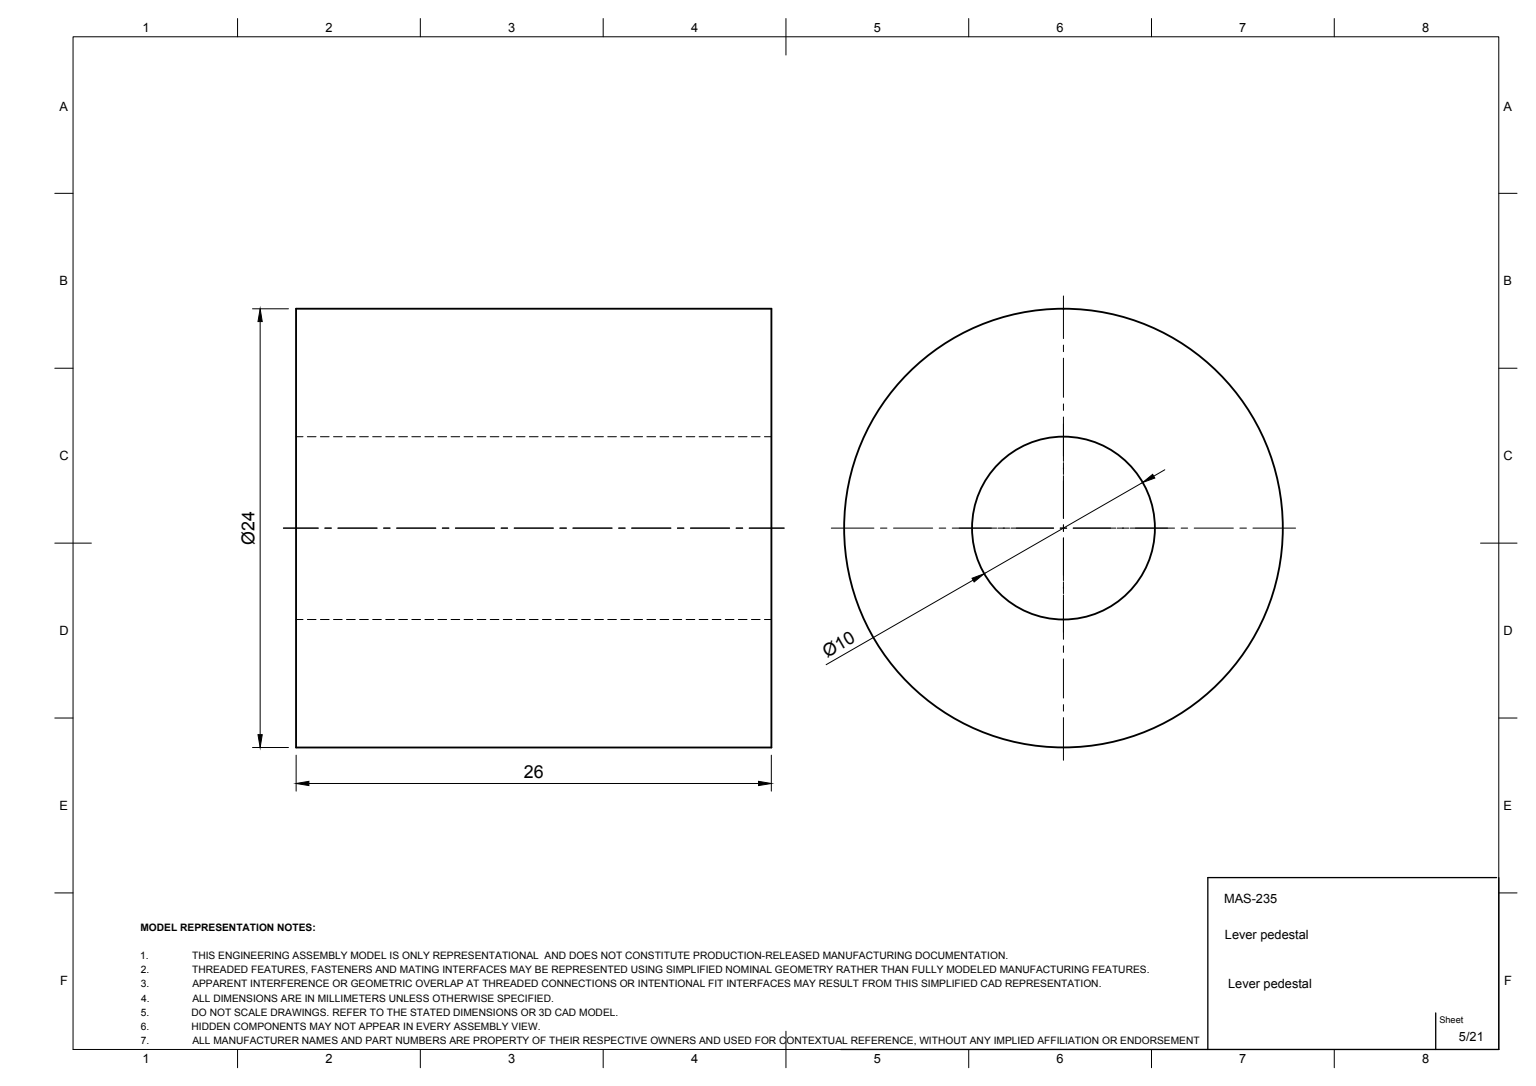
ISO-10303-21;
HEADER;
/* Generated by software containing ST-Developer
 * from STEP Tools, Inc. (www.steptools.com) 
 */

FILE_DESCRIPTION(
/* description */ ('Independent Whitworth quick-return mechanism. Crank radius40, ground-
center spacing80, lever180, connecting rod160, output guide X200. Nomi
nal stroke180 and long/short phase ratio2. Retained guide rods, replac
eable bearing sleeves and captured sliding shoe. No load or production
 rating assigned.'),
/* implementation_level */ '2;1');

FILE_NAME(
/* name */ 'Lever pedestal.step',
/* time_stamp */ '2026-11-09T18:22:56-08:00',
/* author */ (''),
/* organization */ (''),
/* preprocessor_version */ 'ST-DEVELOPER v20.2',
/* originating_system */ 'Autodesk Translation Framework v15.17.0.0',
/* authorisation */ '');

FILE_SCHEMA (('AUTOMOTIVE_DESIGN { 1 0 10303 214 3 1 1 }'));
ENDSEC;

DATA;
#10=MECHANICAL_DESIGN_GEOMETRIC_PRESENTATION_REPRESENTATION('',(#221),#4388);
#181=SHAPE_REPRESENTATION_RELATIONSHIP('SRR','None',#4480,#201);
#201=ADVANCED_BREP_SHAPE_REPRESENTATION('',(#241),#4370);
#221=STYLED_ITEM('',(#4588),#241);
#241=MANIFOLD_SOLID_BREP('Body1',#2326);
#265=FACE_BOUND('',#573,.T.);
#266=FACE_BOUND('',#575,.T.);
#327=PLANE('',#2595);
#328=PLANE('',#2596);
#417=FACE_OUTER_BOUND('',#570,.T.);
#418=FACE_OUTER_BOUND('',#571,.T.);
#419=FACE_OUTER_BOUND('',#572,.T.);
#420=FACE_OUTER_BOUND('',#574,.T.);
#570=EDGE_LOOP('',(#1642,#1643,#1644,#1645));
#571=EDGE_LOOP('',(#1646,#1647,#1648,#1649));
#572=EDGE_LOOP('',(#1650));
#573=EDGE_LOOP('',(#1651));
#574=EDGE_LOOP('',(#1652));
#575=EDGE_LOOP('',(#1653));
#775=LINE('',#3760,#914);
#776=LINE('',#3766,#915);
#914=VECTOR('',#2965,5.);
#915=VECTOR('',#2972,12.);
#1045=CIRCLE('',#2590,5.);
#1046=CIRCLE('',#2591,5.);
#1047=CIRCLE('',#2593,12.);
#1048=CIRCLE('',#2594,12.);
#1175=VERTEX_POINT('',#3757);
#1176=VERTEX_POINT('',#3759);
#1177=VERTEX_POINT('',#3763);
#1178=VERTEX_POINT('',#3765);
#1357=EDGE_CURVE('',#1175,#1175,#1045,.T.);
#1358=EDGE_CURVE('',#1175,#1176,#775,.T.);
#1359=EDGE_CURVE('',#1176,#1176,#1046,.T.);
#1360=EDGE_CURVE('',#1177,#1177,#1047,.T.);
#1361=EDGE_CURVE('',#1177,#1178,#776,.T.);
#1362=EDGE_CURVE('',#1178,#1178,#1048,.T.);
#1642=ORIENTED_EDGE('',*,*,#1357,.F.);
#1643=ORIENTED_EDGE('',*,*,#1358,.T.);
#1644=ORIENTED_EDGE('',*,*,#1359,.T.);
#1645=ORIENTED_EDGE('',*,*,#1358,.F.);
#1646=ORIENTED_EDGE('',*,*,#1360,.F.);
#1647=ORIENTED_EDGE('',*,*,#1361,.T.);
#1648=ORIENTED_EDGE('',*,*,#1362,.T.);
#1649=ORIENTED_EDGE('',*,*,#1361,.F.);
#1650=ORIENTED_EDGE('',*,*,#1360,.T.);
#1651=ORIENTED_EDGE('',*,*,#1357,.T.);
#1652=ORIENTED_EDGE('',*,*,#1362,.F.);
#1653=ORIENTED_EDGE('',*,*,#1359,.F.);
#2120=CYLINDRICAL_SURFACE('',#2589,5.);
#2121=CYLINDRICAL_SURFACE('',#2592,12.);
#2189=ADVANCED_FACE('',(#417),#2120,.F.);
#2190=ADVANCED_FACE('',(#418),#2121,.T.);
#2191=ADVANCED_FACE('',(#419,#265),#327,.T.);
#2192=ADVANCED_FACE('',(#420,#266),#328,.F.);
#2326=CLOSED_SHELL('',(#2189,#2190,#2191,#2192));
#2588=AXIS2_PLACEMENT_3D('',#3755,#2959,#2960);
#2589=AXIS2_PLACEMENT_3D('',#3756,#2961,#2962);
#2590=AXIS2_PLACEMENT_3D('',#3758,#2963,#2964);
#2591=AXIS2_PLACEMENT_3D('',#3761,#2966,#2967);
#2592=AXIS2_PLACEMENT_3D('',#3762,#2968,#2969);
#2593=AXIS2_PLACEMENT_3D('',#3764,#2970,#2971);
#2594=AXIS2_PLACEMENT_3D('',#3767,#2973,#2974);
#2595=AXIS2_PLACEMENT_3D('',#3768,#2975,#2976);
#2596=AXIS2_PLACEMENT_3D('',#3769,#2977,#2978);
#2959=DIRECTION('axis',(0.,0.,1.));
#2960=DIRECTION('refdir',(1.,0.,0.));
#2961=DIRECTION('center_axis',(0.,0.,1.));
#2962=DIRECTION('ref_axis',(1.,0.,0.));
#2963=DIRECTION('center_axis',(0.,0.,-1.));
#2964=DIRECTION('ref_axis',(1.,0.,0.));
#2965=DIRECTION('',(0.,0.,-1.));
#2966=DIRECTION('center_axis',(0.,0.,-1.));
#2967=DIRECTION('ref_axis',(1.,0.,0.));
#2968=DIRECTION('center_axis',(0.,0.,1.));
#2969=DIRECTION('ref_axis',(1.,0.,0.));
#2970=DIRECTION('center_axis',(0.,0.,1.));
#2971=DIRECTION('ref_axis',(1.,0.,0.));
#2972=DIRECTION('',(0.,0.,-1.));
#2973=DIRECTION('center_axis',(0.,0.,1.));
#2974=DIRECTION('ref_axis',(1.,0.,0.));
#2975=DIRECTION('center_axis',(0.,0.,1.));
#2976=DIRECTION('ref_axis',(1.,0.,0.));
#2977=DIRECTION('center_axis',(0.,0.,1.));
#2978=DIRECTION('ref_axis',(1.,0.,0.));
#3755=CARTESIAN_POINT('',(0.,0.,0.));
#3756=CARTESIAN_POINT('Origin',(0.,0.,0.));
#3757=CARTESIAN_POINT('',(-5.,-6.12323399573677E-16,26.));
#3758=CARTESIAN_POINT('Origin',(0.,0.,26.));
#3759=CARTESIAN_POINT('',(-5.,-6.12323399573677E-16,0.));
#3760=CARTESIAN_POINT('',(-5.,-6.12323399573677E-16,0.));
#3761=CARTESIAN_POINT('Origin',(0.,0.,0.));
#3762=CARTESIAN_POINT('Origin',(0.,0.,0.));
#3763=CARTESIAN_POINT('',(-12.,-1.46957615897682E-15,26.));
#3764=CARTESIAN_POINT('Origin',(0.,0.,26.));
#3765=CARTESIAN_POINT('',(-12.,-1.46957615897682E-15,0.));
#3766=CARTESIAN_POINT('',(-12.,-1.46957615897682E-15,0.));
#3767=CARTESIAN_POINT('Origin',(0.,0.,0.));
#3768=CARTESIAN_POINT('Origin',(0.,0.,26.));
#3769=CARTESIAN_POINT('Origin',(0.,0.,0.));
#4348=UNCERTAINTY_MEASURE_WITH_UNIT(LENGTH_MEASURE(0.01),#4389,
'DISTANCE_ACCURACY_VALUE',
'Maximum model space distance between geometric entities at asserted c
onnectivities');
#4366=UNCERTAINTY_MEASURE_WITH_UNIT(LENGTH_MEASURE(0.01),#4389,
'DISTANCE_ACCURACY_VALUE',
'Maximum model space distance between geometric entities at asserted c
onnectivities');
#4370=(
GEOMETRIC_REPRESENTATION_CONTEXT(3)
GLOBAL_UNCERTAINTY_ASSIGNED_CONTEXT((#4348))
GLOBAL_UNIT_ASSIGNED_CONTEXT((#4389,#4391,#4392))
REPRESENTATION_CONTEXT('','3D')
);
#4388=(
GEOMETRIC_REPRESENTATION_CONTEXT(3)
GLOBAL_UNCERTAINTY_ASSIGNED_CONTEXT((#4366))
GLOBAL_UNIT_ASSIGNED_CONTEXT((#4389,#4391,#4392))
REPRESENTATION_CONTEXT('','3D')
);
#4389=(
LENGTH_UNIT()
NAMED_UNIT(*)
SI_UNIT(.MILLI.,.METRE.)
);
#4391=(
NAMED_UNIT(*)
PLANE_ANGLE_UNIT()
SI_UNIT($,.RADIAN.)
);
#4392=(
NAMED_UNIT(*)
SI_UNIT($,.STERADIAN.)
SOLID_ANGLE_UNIT()
);
#4396=SHAPE_DEFINITION_REPRESENTATION(#4417,#4480);
#4417=PRODUCT_DEFINITION_SHAPE('',$,#4502);
#4480=SHAPE_REPRESENTATION('',(#2588),#4370);
#4498=PRODUCT_DEFINITION_CONTEXT('part definition',#4563,'design');
#4502=PRODUCT_DEFINITION('Lever pedestal','Lever pedestal',#4523,#4498);
#4523=PRODUCT_DEFINITION_FORMATION('',$,#4568);
#4563=APPLICATION_CONTEXT(
'Core Data for Automotive Mechanical Design Process');
#4564=PRODUCT_CONTEXT('part definition',#4563,'mechanical');
#4568=PRODUCT('Lever pedestal','Lever pedestal',$,(#4564));
#4588=PRESENTATION_STYLE_ASSIGNMENT((#4602));
#4602=SURFACE_STYLE_USAGE(.BOTH.,#4616);
#4616=SURFACE_SIDE_STYLE('',(#4630));
#4630=SURFACE_STYLE_FILL_AREA(#4644);
#4644=FILL_AREA_STYLE('Support gray',(#4658));
#4658=FILL_AREA_STYLE_COLOUR('Support gray',#4672);
#4672=COLOUR_RGB('Support gray',0.407843137254902,0.447058823529412,0.498039215686275);
ENDSEC;
END-ISO-10303-21;
